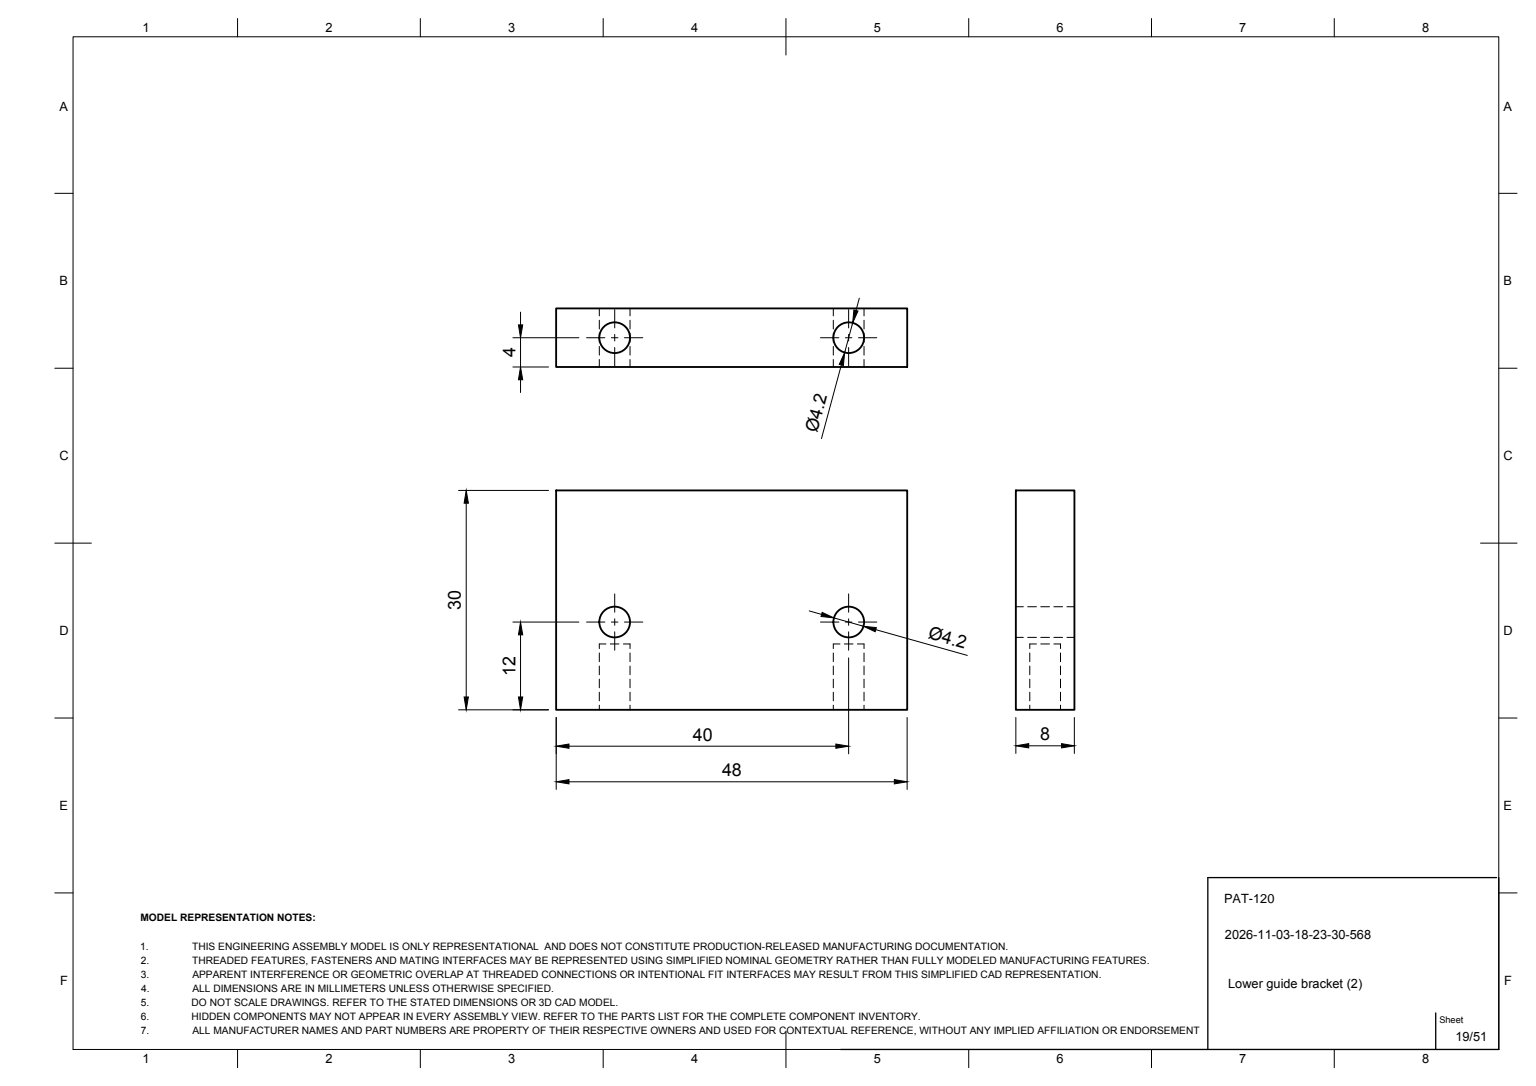
ISO-10303-21;
HEADER;
/* Generated by software containing ST-Developer
 * from STEP Tools, Inc. (www.steptools.com) 
 */

FILE_DESCRIPTION(
/* description */ ('Vibration shaker table dummy'),
/* implementation_level */ '2;1');

FILE_NAME(
/* name */ 'Lower guide bracket (2).step',
/* time_stamp */ '2026-10-27T10:55:14-07:00',
/* author */ (''),
/* organization */ (''),
/* preprocessor_version */ 'ST-DEVELOPER v20.2',
/* originating_system */ 'Autodesk Translation Framework v15.17.0.0',
/* authorisation */ '');

FILE_SCHEMA (('AUTOMOTIVE_DESIGN { 1 0 10303 214 3 1 1 }'));
ENDSEC;

DATA;
#10=MECHANICAL_DESIGN_GEOMETRIC_PRESENTATION_REPRESENTATION('',(#700),#22394);
#608=SHAPE_REPRESENTATION_RELATIONSHIP('SRR','None',#22654,#654);
#654=ADVANCED_BREP_SHAPE_REPRESENTATION('',(#746),#22360);
#700=STYLED_ITEM('',(#22940),#746);
#746=MANIFOLD_SOLID_BREP('Body1',#9218);
#891=FACE_BOUND('',#2120,.T.);
#892=FACE_BOUND('',#2121,.T.);
#893=FACE_BOUND('',#2124,.T.);
#894=FACE_BOUND('',#2125,.T.);
#895=FACE_BOUND('',#2129,.T.);
#896=FACE_BOUND('',#2130,.T.);
#1148=PLANE('',#10084);
#1149=PLANE('',#10088);
#1150=PLANE('',#10095);
#1151=PLANE('',#10096);
#1152=PLANE('',#10097);
#1153=PLANE('',#10098);
#1154=PLANE('',#10099);
#1155=PLANE('',#10100);
#1499=FACE_OUTER_BOUND('',#2113,.T.);
#1500=FACE_OUTER_BOUND('',#2114,.T.);
#1501=FACE_OUTER_BOUND('',#2115,.T.);
#1502=FACE_OUTER_BOUND('',#2116,.T.);
#1503=FACE_OUTER_BOUND('',#2117,.T.);
#1504=FACE_OUTER_BOUND('',#2118,.T.);
#1505=FACE_OUTER_BOUND('',#2119,.T.);
#1506=FACE_OUTER_BOUND('',#2122,.T.);
#1507=FACE_OUTER_BOUND('',#2123,.T.);
#1508=FACE_OUTER_BOUND('',#2126,.T.);
#1509=FACE_OUTER_BOUND('',#2127,.T.);
#1510=FACE_OUTER_BOUND('',#2128,.T.);
#2113=EDGE_LOOP('',(#6978,#6979,#6980,#6981));
#2114=EDGE_LOOP('',(#6982));
#2115=EDGE_LOOP('',(#6983,#6984,#6985,#6986));
#2116=EDGE_LOOP('',(#6987));
#2117=EDGE_LOOP('',(#6988,#6989,#6990,#6991));
#2118=EDGE_LOOP('',(#6992,#6993,#6994,#6995));
#2119=EDGE_LOOP('',(#6996,#6997,#6998,#6999));
#2120=EDGE_LOOP('',(#7000));
#2121=EDGE_LOOP('',(#7001));
#2122=EDGE_LOOP('',(#7002,#7003,#7004,#7005));
#2123=EDGE_LOOP('',(#7006,#7007,#7008,#7009));
#2124=EDGE_LOOP('',(#7010));
#2125=EDGE_LOOP('',(#7011));
#2126=EDGE_LOOP('',(#7012,#7013,#7014,#7015));
#2127=EDGE_LOOP('',(#7016,#7017,#7018,#7019));
#2128=EDGE_LOOP('',(#7020,#7021,#7022,#7023));
#2129=EDGE_LOOP('',(#7024));
#2130=EDGE_LOOP('',(#7025));
#2838=LINE('',#17605,#3457);
#2839=LINE('',#17612,#3458);
#2840=LINE('',#17619,#3459);
#2841=LINE('',#17625,#3460);
#2842=LINE('',#17630,#3461);
#2843=LINE('',#17632,#3462);
#2844=LINE('',#17634,#3463);
#2845=LINE('',#17635,#3464);
#2846=LINE('',#17638,#3465);
#2847=LINE('',#17640,#3466);
#2848=LINE('',#17641,#3467);
#2849=LINE('',#17644,#3468);
#2850=LINE('',#17646,#3469);
#2851=LINE('',#17647,#3470);
#2852=LINE('',#17649,#3471);
#2853=LINE('',#17650,#3472);
#3457=VECTOR('',#11812,0.21);
#3458=VECTOR('',#11821,0.21);
#3459=VECTOR('',#11830,0.21);
#3460=VECTOR('',#11837,0.21);
#3461=VECTOR('',#11842,1.);
#3462=VECTOR('',#11843,1.);
#3463=VECTOR('',#11844,1.);
#3464=VECTOR('',#11845,1.);
#3465=VECTOR('',#11848,1.);
#3466=VECTOR('',#11849,1.);
#3467=VECTOR('',#11850,1.);
#3468=VECTOR('',#11853,1.);
#3469=VECTOR('',#11854,1.);
#3470=VECTOR('',#11855,1.);
#3471=VECTOR('',#11858,1.);
#3472=VECTOR('',#11859,1.);
#4008=CIRCLE('',#10082,0.21);
#4009=CIRCLE('',#10083,0.21);
#4010=CIRCLE('',#10086,0.21);
#4011=CIRCLE('',#10087,0.21);
#4012=CIRCLE('',#10090,0.21);
#4013=CIRCLE('',#10091,0.21);
#4014=CIRCLE('',#10093,0.21);
#4015=CIRCLE('',#10094,0.21);
#4611=VERTEX_POINT('',#17602);
#4612=VERTEX_POINT('',#17604);
#4613=VERTEX_POINT('',#17609);
#4614=VERTEX_POINT('',#17611);
#4615=VERTEX_POINT('',#17616);
#4616=VERTEX_POINT('',#17618);
#4617=VERTEX_POINT('',#17622);
#4618=VERTEX_POINT('',#17624);
#4619=VERTEX_POINT('',#17628);
#4620=VERTEX_POINT('',#17629);
#4621=VERTEX_POINT('',#17631);
#4622=VERTEX_POINT('',#17633);
#4623=VERTEX_POINT('',#17637);
#4624=VERTEX_POINT('',#17639);
#4625=VERTEX_POINT('',#17643);
#4626=VERTEX_POINT('',#17645);
#5482=EDGE_CURVE('',#4611,#4611,#4008,.T.);
#5483=EDGE_CURVE('',#4611,#4612,#2838,.T.);
#5484=EDGE_CURVE('',#4612,#4612,#4009,.T.);
#5485=EDGE_CURVE('',#4613,#4613,#4010,.T.);
#5486=EDGE_CURVE('',#4613,#4614,#2839,.T.);
#5487=EDGE_CURVE('',#4614,#4614,#4011,.T.);
#5488=EDGE_CURVE('',#4615,#4615,#4012,.T.);
#5489=EDGE_CURVE('',#4615,#4616,#2840,.T.);
#5490=EDGE_CURVE('',#4616,#4616,#4013,.T.);
#5491=EDGE_CURVE('',#4617,#4617,#4014,.T.);
#5492=EDGE_CURVE('',#4617,#4618,#2841,.T.);
#5493=EDGE_CURVE('',#4618,#4618,#4015,.T.);
#5494=EDGE_CURVE('',#4619,#4620,#2842,.T.);
#5495=EDGE_CURVE('',#4620,#4621,#2843,.T.);
#5496=EDGE_CURVE('',#4622,#4621,#2844,.T.);
#5497=EDGE_CURVE('',#4619,#4622,#2845,.T.);
#5498=EDGE_CURVE('',#4623,#4619,#2846,.T.);
#5499=EDGE_CURVE('',#4624,#4622,#2847,.T.);
#5500=EDGE_CURVE('',#4623,#4624,#2848,.T.);
#5501=EDGE_CURVE('',#4625,#4623,#2849,.T.);
#5502=EDGE_CURVE('',#4626,#4624,#2850,.T.);
#5503=EDGE_CURVE('',#4625,#4626,#2851,.T.);
#5504=EDGE_CURVE('',#4620,#4625,#2852,.T.);
#5505=EDGE_CURVE('',#4621,#4626,#2853,.T.);
#6978=ORIENTED_EDGE('',*,*,#5482,.F.);
#6979=ORIENTED_EDGE('',*,*,#5483,.T.);
#6980=ORIENTED_EDGE('',*,*,#5484,.T.);
#6981=ORIENTED_EDGE('',*,*,#5483,.F.);
#6982=ORIENTED_EDGE('',*,*,#5484,.F.);
#6983=ORIENTED_EDGE('',*,*,#5485,.F.);
#6984=ORIENTED_EDGE('',*,*,#5486,.T.);
#6985=ORIENTED_EDGE('',*,*,#5487,.T.);
#6986=ORIENTED_EDGE('',*,*,#5486,.F.);
#6987=ORIENTED_EDGE('',*,*,#5487,.F.);
#6988=ORIENTED_EDGE('',*,*,#5488,.F.);
#6989=ORIENTED_EDGE('',*,*,#5489,.T.);
#6990=ORIENTED_EDGE('',*,*,#5490,.F.);
#6991=ORIENTED_EDGE('',*,*,#5489,.F.);
#6992=ORIENTED_EDGE('',*,*,#5491,.F.);
#6993=ORIENTED_EDGE('',*,*,#5492,.T.);
#6994=ORIENTED_EDGE('',*,*,#5493,.F.);
#6995=ORIENTED_EDGE('',*,*,#5492,.F.);
#6996=ORIENTED_EDGE('',*,*,#5494,.T.);
#6997=ORIENTED_EDGE('',*,*,#5495,.T.);
#6998=ORIENTED_EDGE('',*,*,#5496,.F.);
#6999=ORIENTED_EDGE('',*,*,#5497,.F.);
#7000=ORIENTED_EDGE('',*,*,#5490,.T.);
#7001=ORIENTED_EDGE('',*,*,#5493,.T.);
#7002=ORIENTED_EDGE('',*,*,#5498,.T.);
#7003=ORIENTED_EDGE('',*,*,#5497,.T.);
#7004=ORIENTED_EDGE('',*,*,#5499,.F.);
#7005=ORIENTED_EDGE('',*,*,#5500,.F.);
#7006=ORIENTED_EDGE('',*,*,#5501,.T.);
#7007=ORIENTED_EDGE('',*,*,#5500,.T.);
#7008=ORIENTED_EDGE('',*,*,#5502,.F.);
#7009=ORIENTED_EDGE('',*,*,#5503,.F.);
#7010=ORIENTED_EDGE('',*,*,#5488,.T.);
#7011=ORIENTED_EDGE('',*,*,#5491,.T.);
#7012=ORIENTED_EDGE('',*,*,#5504,.T.);
#7013=ORIENTED_EDGE('',*,*,#5503,.T.);
#7014=ORIENTED_EDGE('',*,*,#5505,.F.);
#7015=ORIENTED_EDGE('',*,*,#5495,.F.);
#7016=ORIENTED_EDGE('',*,*,#5505,.T.);
#7017=ORIENTED_EDGE('',*,*,#5502,.T.);
#7018=ORIENTED_EDGE('',*,*,#5499,.T.);
#7019=ORIENTED_EDGE('',*,*,#5496,.T.);
#7020=ORIENTED_EDGE('',*,*,#5504,.F.);
#7021=ORIENTED_EDGE('',*,*,#5494,.F.);
#7022=ORIENTED_EDGE('',*,*,#5498,.F.);
#7023=ORIENTED_EDGE('',*,*,#5501,.F.);
#7024=ORIENTED_EDGE('',*,*,#5482,.T.);
#7025=ORIENTED_EDGE('',*,*,#5485,.T.);
#8574=CYLINDRICAL_SURFACE('',#10081,0.21);
#8575=CYLINDRICAL_SURFACE('',#10085,0.21);
#8576=CYLINDRICAL_SURFACE('',#10089,0.21);
#8577=CYLINDRICAL_SURFACE('',#10092,0.21);
#8864=ADVANCED_FACE('',(#1499),#8574,.F.);
#8865=ADVANCED_FACE('',(#1500),#1148,.F.);
#8866=ADVANCED_FACE('',(#1501),#8575,.F.);
#8867=ADVANCED_FACE('',(#1502),#1149,.F.);
#8868=ADVANCED_FACE('',(#1503),#8576,.F.);
#8869=ADVANCED_FACE('',(#1504),#8577,.F.);
#8870=ADVANCED_FACE('',(#1505,#891,#892),#1150,.T.);
#8871=ADVANCED_FACE('',(#1506),#1151,.T.);
#8872=ADVANCED_FACE('',(#1507,#893,#894),#1152,.T.);
#8873=ADVANCED_FACE('',(#1508),#1153,.T.);
#8874=ADVANCED_FACE('',(#1509),#1154,.T.);
#8875=ADVANCED_FACE('',(#1510,#895,#896),#1155,.F.);
#9218=CLOSED_SHELL('',(#8864,#8865,#8866,#8867,#8868,#8869,#8870,#8871,
#8872,#8873,#8874,#8875));
#10080=AXIS2_PLACEMENT_3D('',#17600,#11806,#11807);
#10081=AXIS2_PLACEMENT_3D('',#17601,#11808,#11809);
#10082=AXIS2_PLACEMENT_3D('',#17603,#11810,#11811);
#10083=AXIS2_PLACEMENT_3D('',#17606,#11813,#11814);
#10084=AXIS2_PLACEMENT_3D('',#17607,#11815,#11816);
#10085=AXIS2_PLACEMENT_3D('',#17608,#11817,#11818);
#10086=AXIS2_PLACEMENT_3D('',#17610,#11819,#11820);
#10087=AXIS2_PLACEMENT_3D('',#17613,#11822,#11823);
#10088=AXIS2_PLACEMENT_3D('',#17614,#11824,#11825);
#10089=AXIS2_PLACEMENT_3D('',#17615,#11826,#11827);
#10090=AXIS2_PLACEMENT_3D('',#17617,#11828,#11829);
#10091=AXIS2_PLACEMENT_3D('',#17620,#11831,#11832);
#10092=AXIS2_PLACEMENT_3D('',#17621,#11833,#11834);
#10093=AXIS2_PLACEMENT_3D('',#17623,#11835,#11836);
#10094=AXIS2_PLACEMENT_3D('',#17626,#11838,#11839);
#10095=AXIS2_PLACEMENT_3D('',#17627,#11840,#11841);
#10096=AXIS2_PLACEMENT_3D('',#17636,#11846,#11847);
#10097=AXIS2_PLACEMENT_3D('',#17642,#11851,#11852);
#10098=AXIS2_PLACEMENT_3D('',#17648,#11856,#11857);
#10099=AXIS2_PLACEMENT_3D('',#17651,#11860,#11861);
#10100=AXIS2_PLACEMENT_3D('',#17652,#11862,#11863);
#11806=DIRECTION('axis',(0.,0.,1.));
#11807=DIRECTION('refdir',(1.,0.,0.));
#11808=DIRECTION('center_axis',(0.,0.,1.));
#11809=DIRECTION('ref_axis',(1.,0.,0.));
#11810=DIRECTION('center_axis',(0.,0.,1.));
#11811=DIRECTION('ref_axis',(1.,0.,0.));
#11812=DIRECTION('',(0.,0.,1.));
#11813=DIRECTION('center_axis',(0.,0.,1.));
#11814=DIRECTION('ref_axis',(1.,0.,0.));
#11815=DIRECTION('center_axis',(0.,0.,1.));
#11816=DIRECTION('ref_axis',(1.,0.,0.));
#11817=DIRECTION('center_axis',(0.,0.,1.));
#11818=DIRECTION('ref_axis',(1.,0.,0.));
#11819=DIRECTION('center_axis',(0.,0.,1.));
#11820=DIRECTION('ref_axis',(1.,0.,0.));
#11821=DIRECTION('',(0.,0.,1.));
#11822=DIRECTION('center_axis',(0.,0.,1.));
#11823=DIRECTION('ref_axis',(1.,0.,0.));
#11824=DIRECTION('center_axis',(0.,0.,1.));
#11825=DIRECTION('ref_axis',(1.,0.,0.));
#11826=DIRECTION('center_axis',(0.,1.,0.));
#11827=DIRECTION('ref_axis',(1.,0.,0.));
#11828=DIRECTION('center_axis',(0.,1.,0.));
#11829=DIRECTION('ref_axis',(1.,0.,0.));
#11830=DIRECTION('',(0.,1.,0.));
#11831=DIRECTION('center_axis',(0.,-1.,0.));
#11832=DIRECTION('ref_axis',(1.,0.,0.));
#11833=DIRECTION('center_axis',(0.,1.,0.));
#11834=DIRECTION('ref_axis',(1.,0.,0.));
#11835=DIRECTION('center_axis',(0.,1.,0.));
#11836=DIRECTION('ref_axis',(1.,0.,0.));
#11837=DIRECTION('',(0.,1.,0.));
#11838=DIRECTION('center_axis',(0.,-1.,0.));
#11839=DIRECTION('ref_axis',(1.,0.,0.));
#11840=DIRECTION('center_axis',(0.,1.,0.));
#11841=DIRECTION('ref_axis',(-1.,0.,0.));
#11842=DIRECTION('',(-1.,0.,0.));
#11843=DIRECTION('',(0.,0.,1.));
#11844=DIRECTION('',(-1.,0.,0.));
#11845=DIRECTION('',(0.,0.,1.));
#11846=DIRECTION('center_axis',(1.,0.,0.));
#11847=DIRECTION('ref_axis',(0.,1.,0.));
#11848=DIRECTION('',(0.,1.,0.));
#11849=DIRECTION('',(0.,1.,0.));
#11850=DIRECTION('',(0.,0.,1.));
#11851=DIRECTION('center_axis',(0.,-1.,0.));
#11852=DIRECTION('ref_axis',(1.,0.,0.));
#11853=DIRECTION('',(1.,0.,0.));
#11854=DIRECTION('',(1.,0.,0.));
#11855=DIRECTION('',(0.,0.,1.));
#11856=DIRECTION('center_axis',(-1.,0.,0.));
#11857=DIRECTION('ref_axis',(0.,-1.,0.));
#11858=DIRECTION('',(0.,-1.,0.));
#11859=DIRECTION('',(0.,-1.,0.));
#11860=DIRECTION('center_axis',(0.,0.,1.));
#11861=DIRECTION('ref_axis',(1.,0.,0.));
#11862=DIRECTION('center_axis',(0.,0.,1.));
#11863=DIRECTION('ref_axis',(1.,0.,0.));
#17600=CARTESIAN_POINT('',(0.,0.,0.));
#17601=CARTESIAN_POINT('Origin',(4.4,-1.3,-0.1));
#17602=CARTESIAN_POINT('',(4.19,-1.3,0.));
#17603=CARTESIAN_POINT('Origin',(4.4,-1.3,0.));
#17604=CARTESIAN_POINT('',(4.19,-1.3,0.9));
#17605=CARTESIAN_POINT('',(4.19,-1.3,-0.1));
#17606=CARTESIAN_POINT('Origin',(4.4,-1.3,0.9));
#17607=CARTESIAN_POINT('Origin',(4.4,-1.3,0.9));
#17608=CARTESIAN_POINT('Origin',(7.6,-1.3,-0.1));
#17609=CARTESIAN_POINT('',(7.39,-1.3,0.));
#17610=CARTESIAN_POINT('Origin',(7.6,-1.3,0.));
#17611=CARTESIAN_POINT('',(7.39,-1.3,0.9));
#17612=CARTESIAN_POINT('',(7.39,-1.3,-0.1));
#17613=CARTESIAN_POINT('Origin',(7.6,-1.3,0.9));
#17614=CARTESIAN_POINT('Origin',(7.6,-1.3,0.9));
#17615=CARTESIAN_POINT('Origin',(4.4,-1.8,1.2));
#17616=CARTESIAN_POINT('',(4.19,-1.7,1.2));
#17617=CARTESIAN_POINT('Origin',(4.4,-1.7,1.2));
#17618=CARTESIAN_POINT('',(4.19,-0.9,1.2));
#17619=CARTESIAN_POINT('',(4.19,-1.8,1.2));
#17620=CARTESIAN_POINT('Origin',(4.4,-0.9,1.2));
#17621=CARTESIAN_POINT('Origin',(7.6,-1.8,1.2));
#17622=CARTESIAN_POINT('',(7.39,-1.7,1.2));
#17623=CARTESIAN_POINT('Origin',(7.6,-1.7,1.2));
#17624=CARTESIAN_POINT('',(7.39,-0.9,1.2));
#17625=CARTESIAN_POINT('',(7.39,-1.8,1.2));
#17626=CARTESIAN_POINT('Origin',(7.6,-0.9,1.2));
#17627=CARTESIAN_POINT('Origin',(8.4,-0.9,0.));
#17628=CARTESIAN_POINT('',(8.4,-0.9,0.));
#17629=CARTESIAN_POINT('',(3.6,-0.9,0.));
#17630=CARTESIAN_POINT('',(8.4,-0.9,0.));
#17631=CARTESIAN_POINT('',(3.6,-0.9,3.));
#17632=CARTESIAN_POINT('',(3.6,-0.9,0.));
#17633=CARTESIAN_POINT('',(8.4,-0.9,3.));
#17634=CARTESIAN_POINT('',(8.4,-0.9,3.));
#17635=CARTESIAN_POINT('',(8.4,-0.9,0.));
#17636=CARTESIAN_POINT('Origin',(8.4,-1.7,0.));
#17637=CARTESIAN_POINT('',(8.4,-1.7,0.));
#17638=CARTESIAN_POINT('',(8.4,-1.7,0.));
#17639=CARTESIAN_POINT('',(8.4,-1.7,3.));
#17640=CARTESIAN_POINT('',(8.4,-1.7,3.));
#17641=CARTESIAN_POINT('',(8.4,-1.7,0.));
#17642=CARTESIAN_POINT('Origin',(3.6,-1.7,0.));
#17643=CARTESIAN_POINT('',(3.6,-1.7,0.));
#17644=CARTESIAN_POINT('',(3.6,-1.7,0.));
#17645=CARTESIAN_POINT('',(3.6,-1.7,3.));
#17646=CARTESIAN_POINT('',(3.6,-1.7,3.));
#17647=CARTESIAN_POINT('',(3.6,-1.7,0.));
#17648=CARTESIAN_POINT('Origin',(3.6,-0.9,0.));
#17649=CARTESIAN_POINT('',(3.6,-0.9,0.));
#17650=CARTESIAN_POINT('',(3.6,-0.9,3.));
#17651=CARTESIAN_POINT('Origin',(6.,-1.3,3.));
#17652=CARTESIAN_POINT('Origin',(6.,-1.3,0.));
#22309=UNCERTAINTY_MEASURE_WITH_UNIT(LENGTH_MEASURE(0.001),#22395,
'DISTANCE_ACCURACY_VALUE',
'Maximum model space distance between geometric entities at asserted c
onnectivities');
#22343=UNCERTAINTY_MEASURE_WITH_UNIT(LENGTH_MEASURE(0.001),#22395,
'DISTANCE_ACCURACY_VALUE',
'Maximum model space distance between geometric entities at asserted c
onnectivities');
#22360=(
GEOMETRIC_REPRESENTATION_CONTEXT(3)
GLOBAL_UNCERTAINTY_ASSIGNED_CONTEXT((#22309))
GLOBAL_UNIT_ASSIGNED_CONTEXT((#22395,#22397,#22398))
REPRESENTATION_CONTEXT('','3D')
);
#22394=(
GEOMETRIC_REPRESENTATION_CONTEXT(3)
GLOBAL_UNCERTAINTY_ASSIGNED_CONTEXT((#22343))
GLOBAL_UNIT_ASSIGNED_CONTEXT((#22395,#22397,#22398))
REPRESENTATION_CONTEXT('','3D')
);
#22395=(
LENGTH_UNIT()
NAMED_UNIT(*)
SI_UNIT(.CENTI.,.METRE.)
);
#22397=(
NAMED_UNIT(*)
PLANE_ANGLE_UNIT()
SI_UNIT($,.RADIAN.)
);
#22398=(
NAMED_UNIT(*)
SI_UNIT($,.STERADIAN.)
SOLID_ANGLE_UNIT()
);
#22415=SHAPE_DEFINITION_REPRESENTATION(#22465,#22654);
#22465=PRODUCT_DEFINITION_SHAPE('',$,#22705);
#22654=SHAPE_REPRESENTATION('',(#10080),#22360);
#22688=PRODUCT_DEFINITION_CONTEXT('part definition',#22840,'design');
#22705=PRODUCT_DEFINITION('Lower guide bracket (2)',
'Lower guide bracket (2)',#22755,#22688);
#22755=PRODUCT_DEFINITION_FORMATION('',$,#22858);
#22840=APPLICATION_CONTEXT(
'Core Data for Automotive Mechanical Design Process');
#22841=PRODUCT_CONTEXT('part definition',#22840,'mechanical');
#22858=PRODUCT('Lower guide bracket (2)','Lower guide bracket (2)',
'Lower guide bracket (2)',(#22841));
#22934=COLOUR_RGB('Dark Blue',0.08,0.2,0.34);
#22935=FILL_AREA_STYLE_COLOUR('',#22934);
#22936=FILL_AREA_STYLE('',(#22935));
#22937=SURFACE_STYLE_FILL_AREA(#22936);
#22938=SURFACE_SIDE_STYLE('',(#22937));
#22939=SURFACE_STYLE_USAGE(.BOTH.,#22938);
#22940=PRESENTATION_STYLE_ASSIGNMENT((#22939));
ENDSEC;
END-ISO-10303-21;
